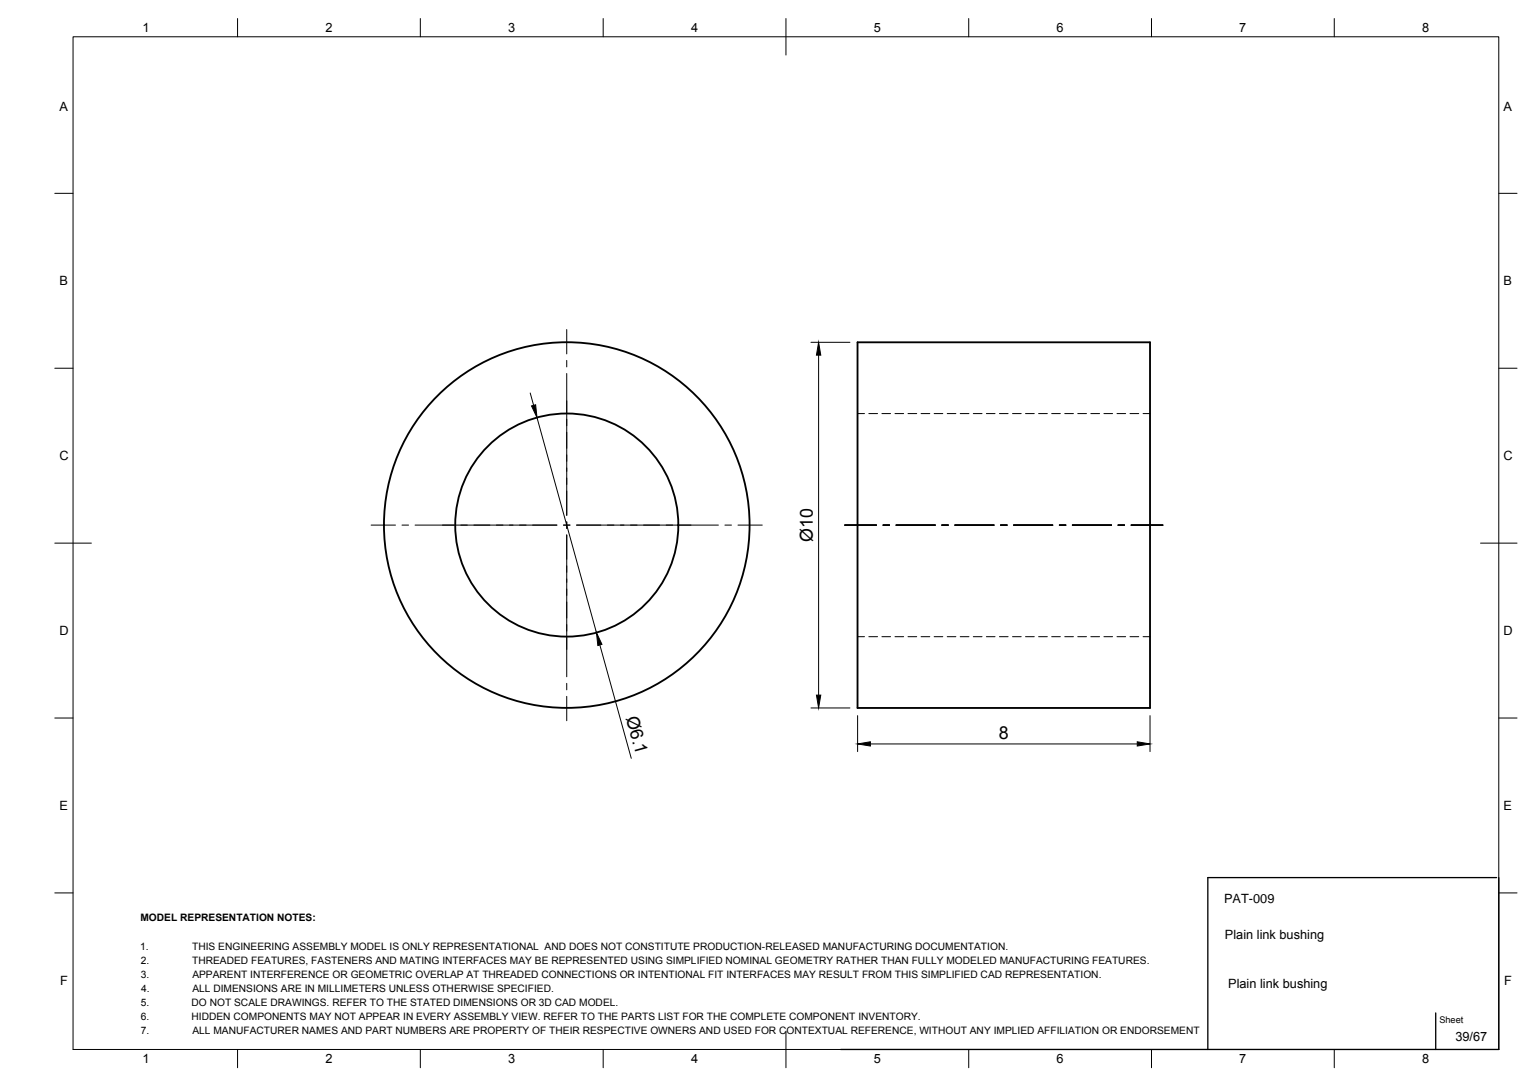
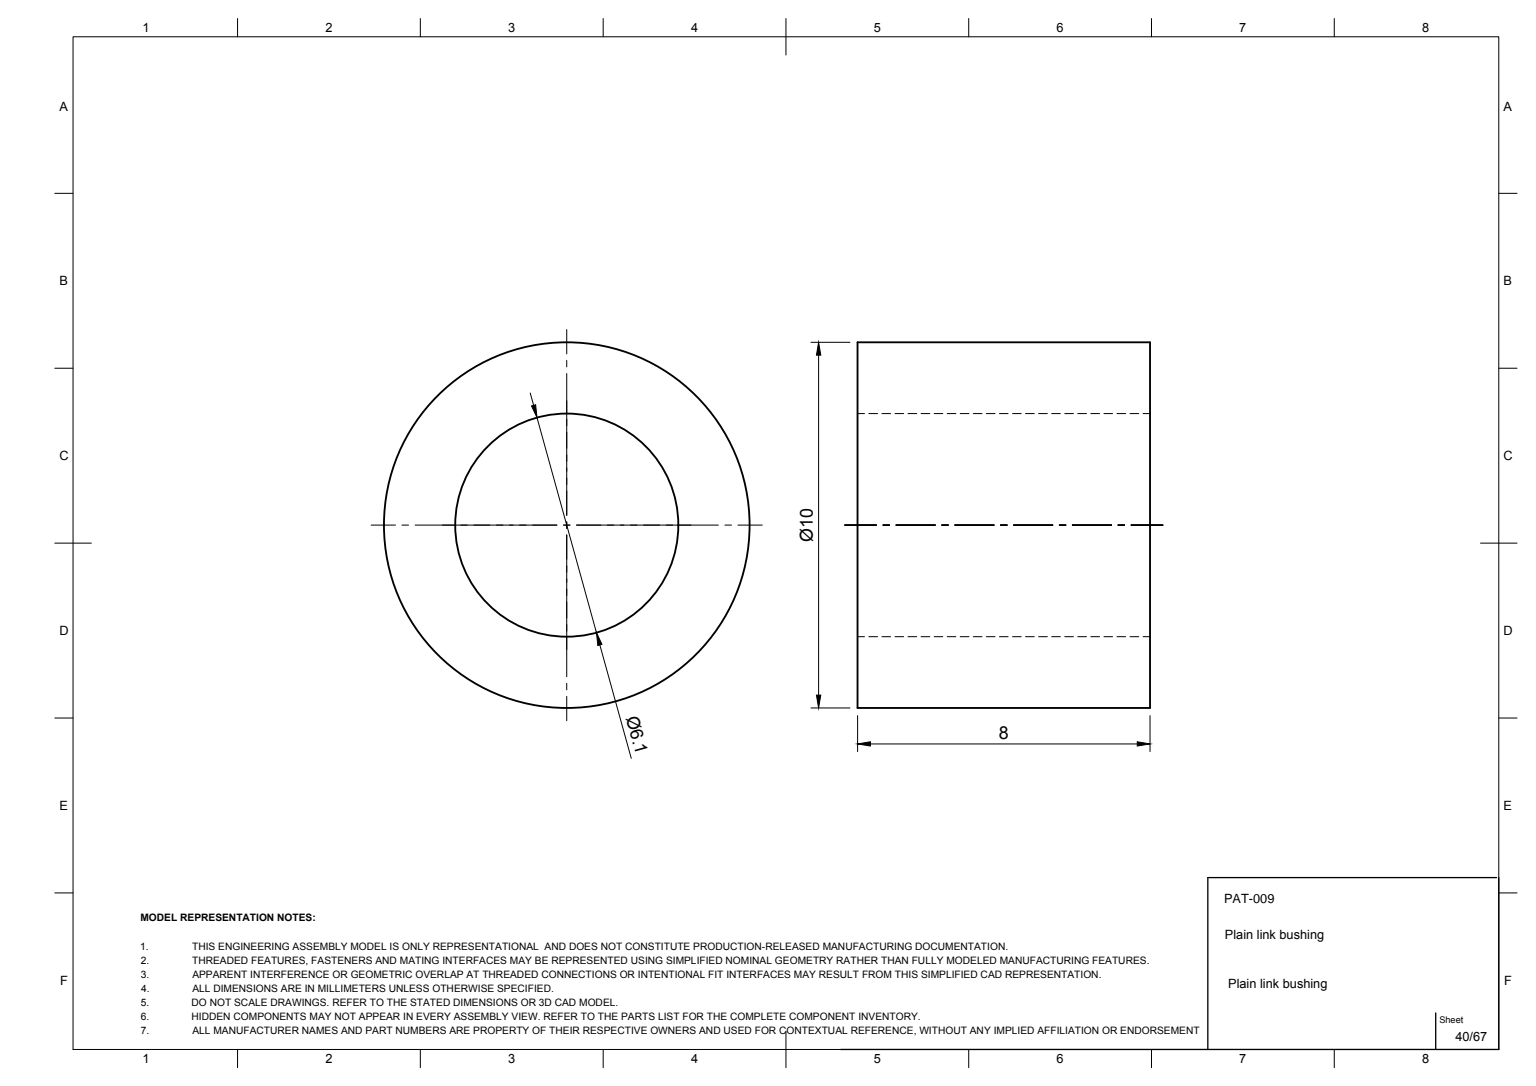
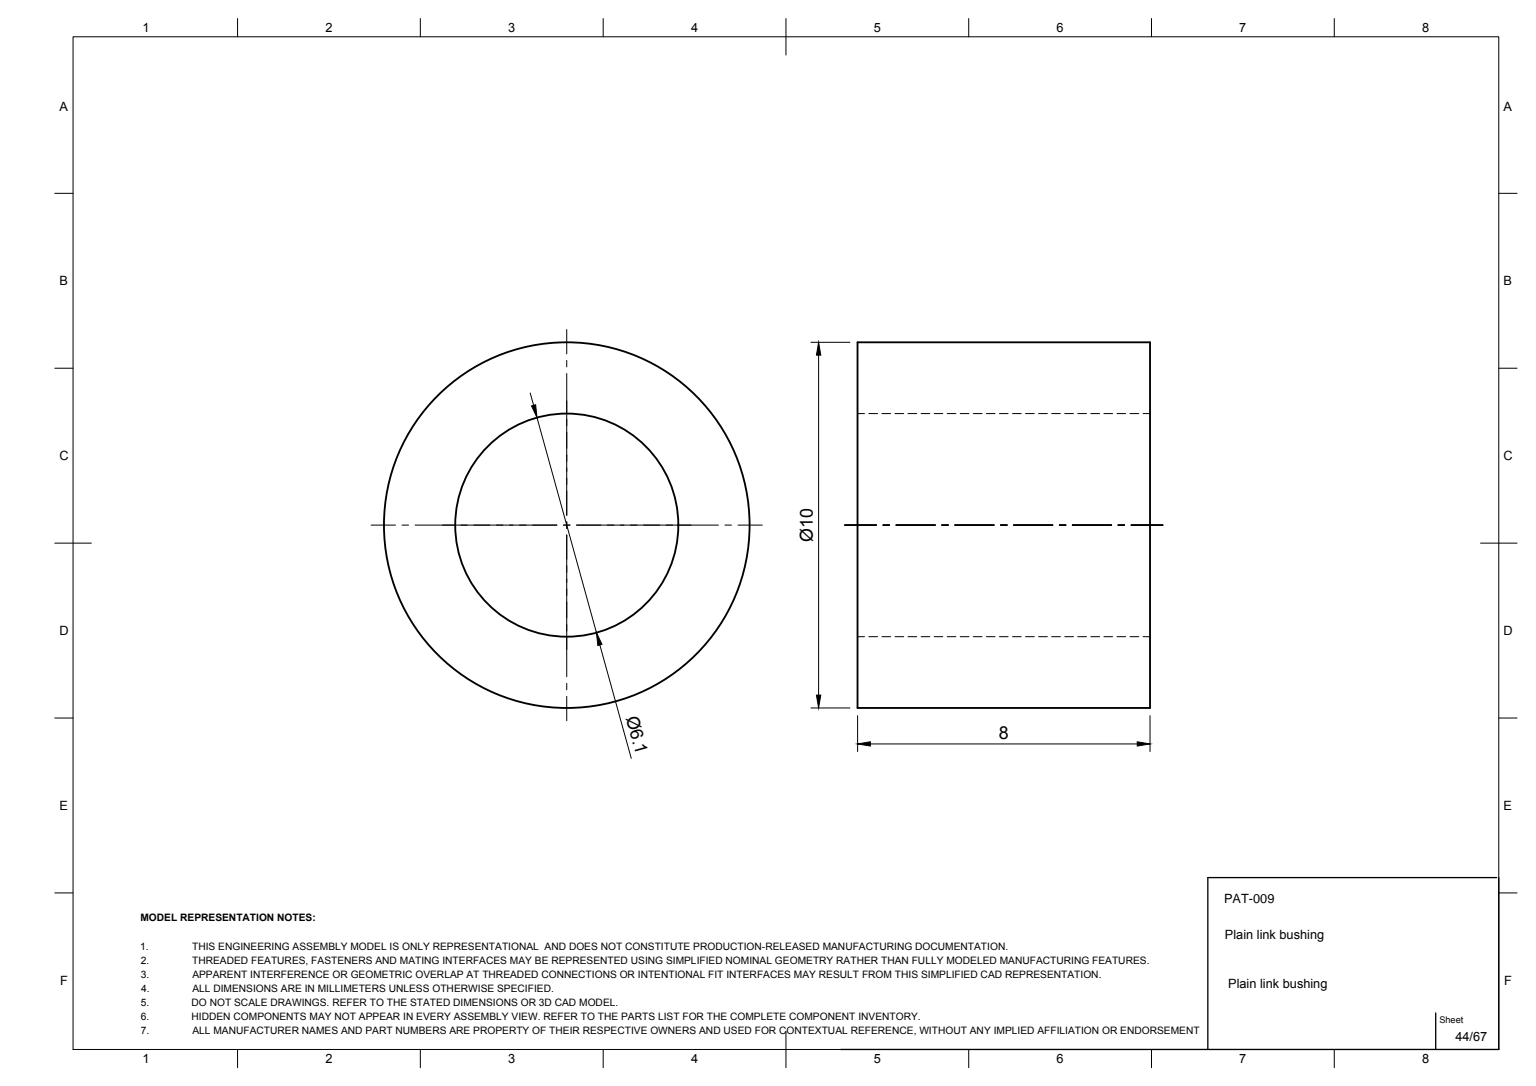
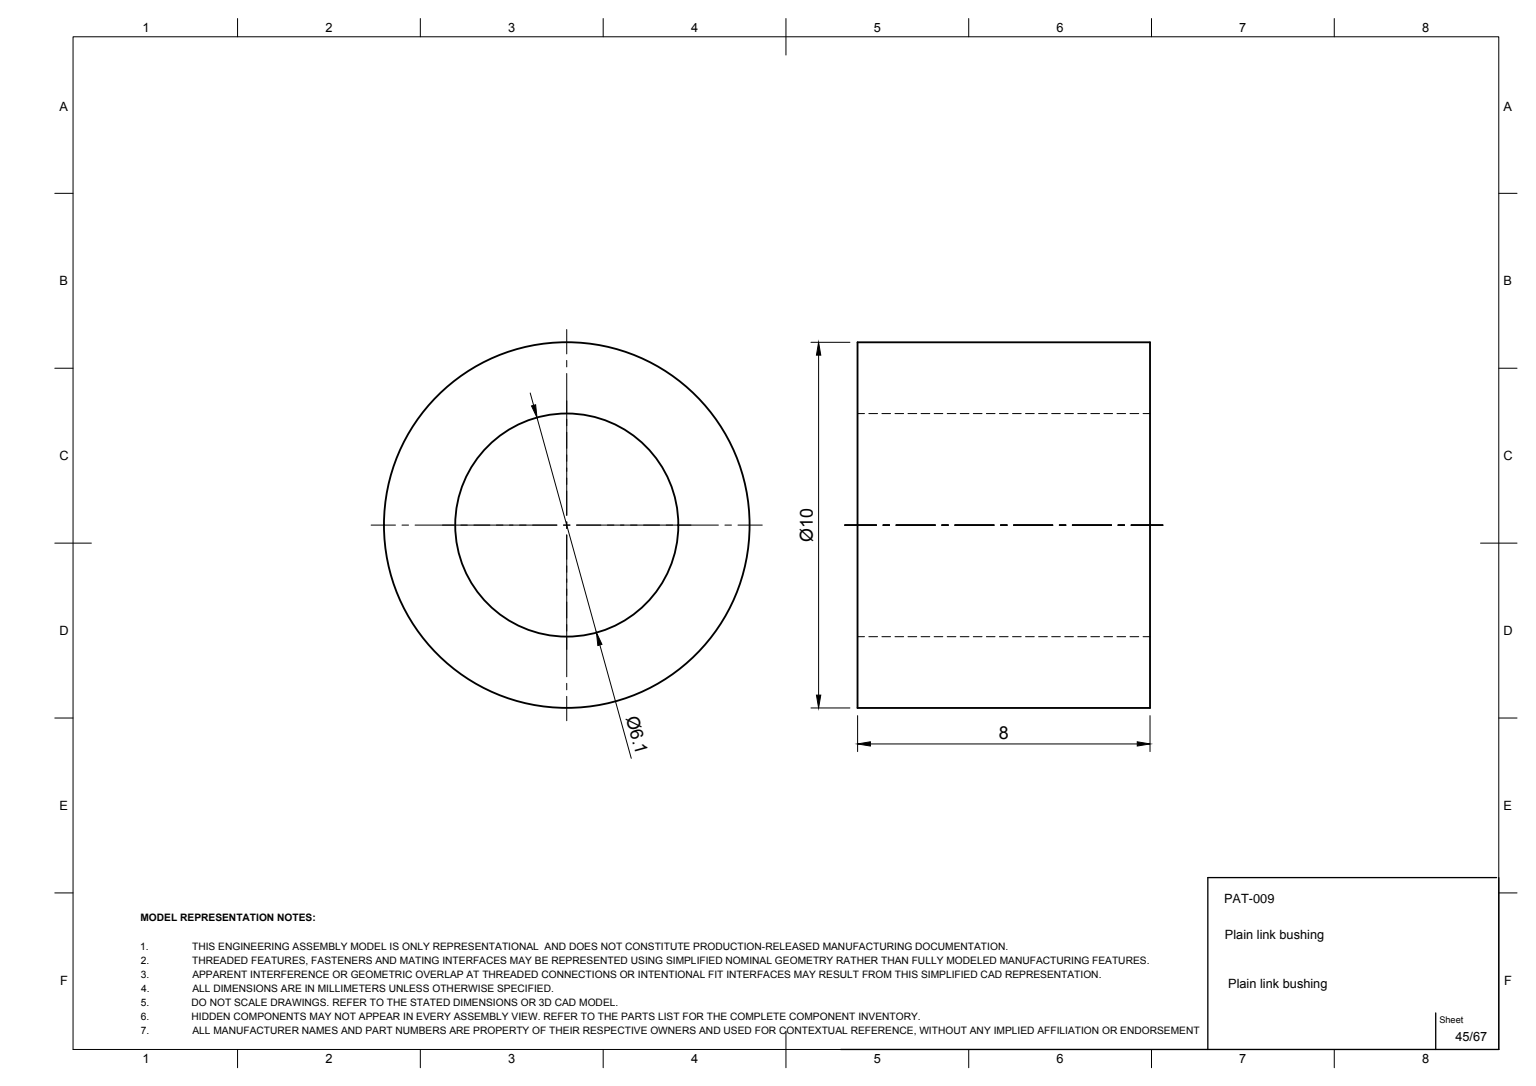
ISO-10303-21;
HEADER;
/* Generated by software containing ST-Developer
 * from STEP Tools, Inc. (www.steptools.com) 
 */

FILE_DESCRIPTION(
/* description */ ('Bell-crank linkage with push rods'),
/* implementation_level */ '2;1');

FILE_NAME(
/* name */ 'Plain link bushing.step',
/* time_stamp */ '2026-10-28T03:25:15-07:00',
/* author */ (''),
/* organization */ (''),
/* preprocessor_version */ 'ST-DEVELOPER v20.2',
/* originating_system */ 'Autodesk Translation Framework v15.17.0.0',
/* authorisation */ '');

FILE_SCHEMA (('AUTOMOTIVE_DESIGN { 1 0 10303 214 3 1 1 }'));
ENDSEC;

DATA;
#10=MECHANICAL_DESIGN_GEOMETRIC_PRESENTATION_REPRESENTATION('',(#644),#16678);
#528=SHAPE_REPRESENTATION_RELATIONSHIP('SRR','None',#16947,#582);
#582=ADVANCED_BREP_SHAPE_REPRESENTATION('',(#704),#16652);
#644=STYLED_ITEM('',(#17284),#704);
#704=MANIFOLD_SOLID_BREP('Body1',#8836);
#862=FACE_BOUND('',#2254,.T.);
#863=FACE_BOUND('',#2256,.T.);
#1147=PLANE('',#10181);
#1148=PLANE('',#10182);
#1592=FACE_OUTER_BOUND('',#2251,.T.);
#1593=FACE_OUTER_BOUND('',#2252,.T.);
#1594=FACE_OUTER_BOUND('',#2253,.T.);
#1595=FACE_OUTER_BOUND('',#2255,.T.);
#2251=EDGE_LOOP('',(#7371,#7372,#7373,#7374));
#2252=EDGE_LOOP('',(#7375,#7376,#7377,#7378));
#2253=EDGE_LOOP('',(#7379));
#2254=EDGE_LOOP('',(#7380));
#2255=EDGE_LOOP('',(#7381));
#2256=EDGE_LOOP('',(#7382));
#2890=LINE('',#15678,#3439);
#2891=LINE('',#15684,#3440);
#3439=VECTOR('',#12434,0.305);
#3440=VECTOR('',#12441,0.5);
#3963=CIRCLE('',#10176,0.305);
#3964=CIRCLE('',#10177,0.305);
#3965=CIRCLE('',#10179,0.5);
#3966=CIRCLE('',#10180,0.5);
#4602=VERTEX_POINT('',#15675);
#4603=VERTEX_POINT('',#15677);
#4604=VERTEX_POINT('',#15681);
#4605=VERTEX_POINT('',#15683);
#5563=EDGE_CURVE('',#4602,#4602,#3963,.T.);
#5564=EDGE_CURVE('',#4602,#4603,#2890,.T.);
#5565=EDGE_CURVE('',#4603,#4603,#3964,.T.);
#5566=EDGE_CURVE('',#4604,#4604,#3965,.T.);
#5567=EDGE_CURVE('',#4604,#4605,#2891,.T.);
#5568=EDGE_CURVE('',#4605,#4605,#3966,.T.);
#7371=ORIENTED_EDGE('',*,*,#5563,.F.);
#7372=ORIENTED_EDGE('',*,*,#5564,.T.);
#7373=ORIENTED_EDGE('',*,*,#5565,.T.);
#7374=ORIENTED_EDGE('',*,*,#5564,.F.);
#7375=ORIENTED_EDGE('',*,*,#5566,.F.);
#7376=ORIENTED_EDGE('',*,*,#5567,.T.);
#7377=ORIENTED_EDGE('',*,*,#5568,.T.);
#7378=ORIENTED_EDGE('',*,*,#5567,.F.);
#7379=ORIENTED_EDGE('',*,*,#5566,.T.);
#7380=ORIENTED_EDGE('',*,*,#5563,.T.);
#7381=ORIENTED_EDGE('',*,*,#5568,.F.);
#7382=ORIENTED_EDGE('',*,*,#5565,.F.);
#8198=CYLINDRICAL_SURFACE('',#10175,0.305);
#8199=CYLINDRICAL_SURFACE('',#10178,0.5);
#8617=ADVANCED_FACE('',(#1592),#8198,.F.);
#8618=ADVANCED_FACE('',(#1593),#8199,.T.);
#8619=ADVANCED_FACE('',(#1594,#862),#1147,.T.);
#8620=ADVANCED_FACE('',(#1595,#863),#1148,.F.);
#8836=CLOSED_SHELL('',(#8617,#8618,#8619,#8620));
#10174=AXIS2_PLACEMENT_3D('',#15673,#12428,#12429);
#10175=AXIS2_PLACEMENT_3D('',#15674,#12430,#12431);
#10176=AXIS2_PLACEMENT_3D('',#15676,#12432,#12433);
#10177=AXIS2_PLACEMENT_3D('',#15679,#12435,#12436);
#10178=AXIS2_PLACEMENT_3D('',#15680,#12437,#12438);
#10179=AXIS2_PLACEMENT_3D('',#15682,#12439,#12440);
#10180=AXIS2_PLACEMENT_3D('',#15685,#12442,#12443);
#10181=AXIS2_PLACEMENT_3D('',#15686,#12444,#12445);
#10182=AXIS2_PLACEMENT_3D('',#15687,#12446,#12447);
#12428=DIRECTION('axis',(0.,0.,1.));
#12429=DIRECTION('refdir',(1.,0.,0.));
#12430=DIRECTION('center_axis',(0.,0.,1.));
#12431=DIRECTION('ref_axis',(1.,0.,0.));
#12432=DIRECTION('center_axis',(0.,0.,-1.));
#12433=DIRECTION('ref_axis',(1.,0.,0.));
#12434=DIRECTION('',(0.,0.,-1.));
#12435=DIRECTION('center_axis',(0.,0.,-1.));
#12436=DIRECTION('ref_axis',(1.,0.,0.));
#12437=DIRECTION('center_axis',(0.,0.,1.));
#12438=DIRECTION('ref_axis',(1.,0.,0.));
#12439=DIRECTION('center_axis',(0.,0.,1.));
#12440=DIRECTION('ref_axis',(1.,0.,0.));
#12441=DIRECTION('',(0.,0.,-1.));
#12442=DIRECTION('center_axis',(0.,0.,1.));
#12443=DIRECTION('ref_axis',(1.,0.,0.));
#12444=DIRECTION('center_axis',(0.,0.,1.));
#12445=DIRECTION('ref_axis',(1.,0.,0.));
#12446=DIRECTION('center_axis',(0.,0.,1.));
#12447=DIRECTION('ref_axis',(1.,0.,0.));
#15673=CARTESIAN_POINT('',(0.,0.,0.));
#15674=CARTESIAN_POINT('Origin',(0.,2.,8.8));
#15675=CARTESIAN_POINT('',(-0.305,2.,9.6));
#15676=CARTESIAN_POINT('Origin',(0.,2.,9.6));
#15677=CARTESIAN_POINT('',(-0.305,2.,8.8));
#15678=CARTESIAN_POINT('',(-0.305,2.,8.8));
#15679=CARTESIAN_POINT('Origin',(0.,2.,8.8));
#15680=CARTESIAN_POINT('Origin',(0.,2.,8.8));
#15681=CARTESIAN_POINT('',(-0.5,2.,9.6));
#15682=CARTESIAN_POINT('Origin',(0.,2.,9.6));
#15683=CARTESIAN_POINT('',(-0.5,2.,8.8));
#15684=CARTESIAN_POINT('',(-0.5,2.,8.8));
#15685=CARTESIAN_POINT('Origin',(0.,2.,8.8));
#15686=CARTESIAN_POINT('Origin',(0.,2.,9.6));
#15687=CARTESIAN_POINT('Origin',(0.,2.,8.8));
#16588=UNCERTAINTY_MEASURE_WITH_UNIT(LENGTH_MEASURE(0.001),#16679,
'DISTANCE_ACCURACY_VALUE',
'Maximum model space distance between geometric entities at asserted c
onnectivities');
#16614=UNCERTAINTY_MEASURE_WITH_UNIT(LENGTH_MEASURE(0.001),#16679,
'DISTANCE_ACCURACY_VALUE',
'Maximum model space distance between geometric entities at asserted c
onnectivities');
#16652=(
GEOMETRIC_REPRESENTATION_CONTEXT(3)
GLOBAL_UNCERTAINTY_ASSIGNED_CONTEXT((#16588))
GLOBAL_UNIT_ASSIGNED_CONTEXT((#16679,#16681,#16682))
REPRESENTATION_CONTEXT('','3D')
);
#16678=(
GEOMETRIC_REPRESENTATION_CONTEXT(3)
GLOBAL_UNCERTAINTY_ASSIGNED_CONTEXT((#16614))
GLOBAL_UNIT_ASSIGNED_CONTEXT((#16679,#16681,#16682))
REPRESENTATION_CONTEXT('','3D')
);
#16679=(
LENGTH_UNIT()
NAMED_UNIT(*)
SI_UNIT(.CENTI.,.METRE.)
);
#16681=(
NAMED_UNIT(*)
PLANE_ANGLE_UNIT()
SI_UNIT($,.RADIAN.)
);
#16682=(
NAMED_UNIT(*)
SI_UNIT($,.STERADIAN.)
SOLID_ANGLE_UNIT()
);
#16720=SHAPE_DEFINITION_REPRESENTATION(#16788,#16947);
#16788=PRODUCT_DEFINITION_SHAPE('',$,#17011);
#16947=SHAPE_REPRESENTATION('',(#10174),#16652);
#16973=PRODUCT_DEFINITION_CONTEXT('part definition',#17164,'design');
#17011=PRODUCT_DEFINITION('Plain link bushing','Plain link bushing',#17074,
#16973);
#17074=PRODUCT_DEFINITION_FORMATION('',$,#17203);
#17164=APPLICATION_CONTEXT(
'Core Data for Automotive Mechanical Design Process');
#17165=PRODUCT_CONTEXT('part definition',#17164,'mechanical');
#17203=PRODUCT('Plain link bushing','Plain link bushing',
'Plain link bushing',(#17165));
#17278=COLOUR_RGB('Sky Blue',0.24,0.69,0.87);
#17279=FILL_AREA_STYLE_COLOUR('',#17278);
#17280=FILL_AREA_STYLE('',(#17279));
#17281=SURFACE_STYLE_FILL_AREA(#17280);
#17282=SURFACE_SIDE_STYLE('',(#17281));
#17283=SURFACE_STYLE_USAGE(.BOTH.,#17282);
#17284=PRESENTATION_STYLE_ASSIGNMENT((#17283));
ENDSEC;
END-ISO-10303-21;
